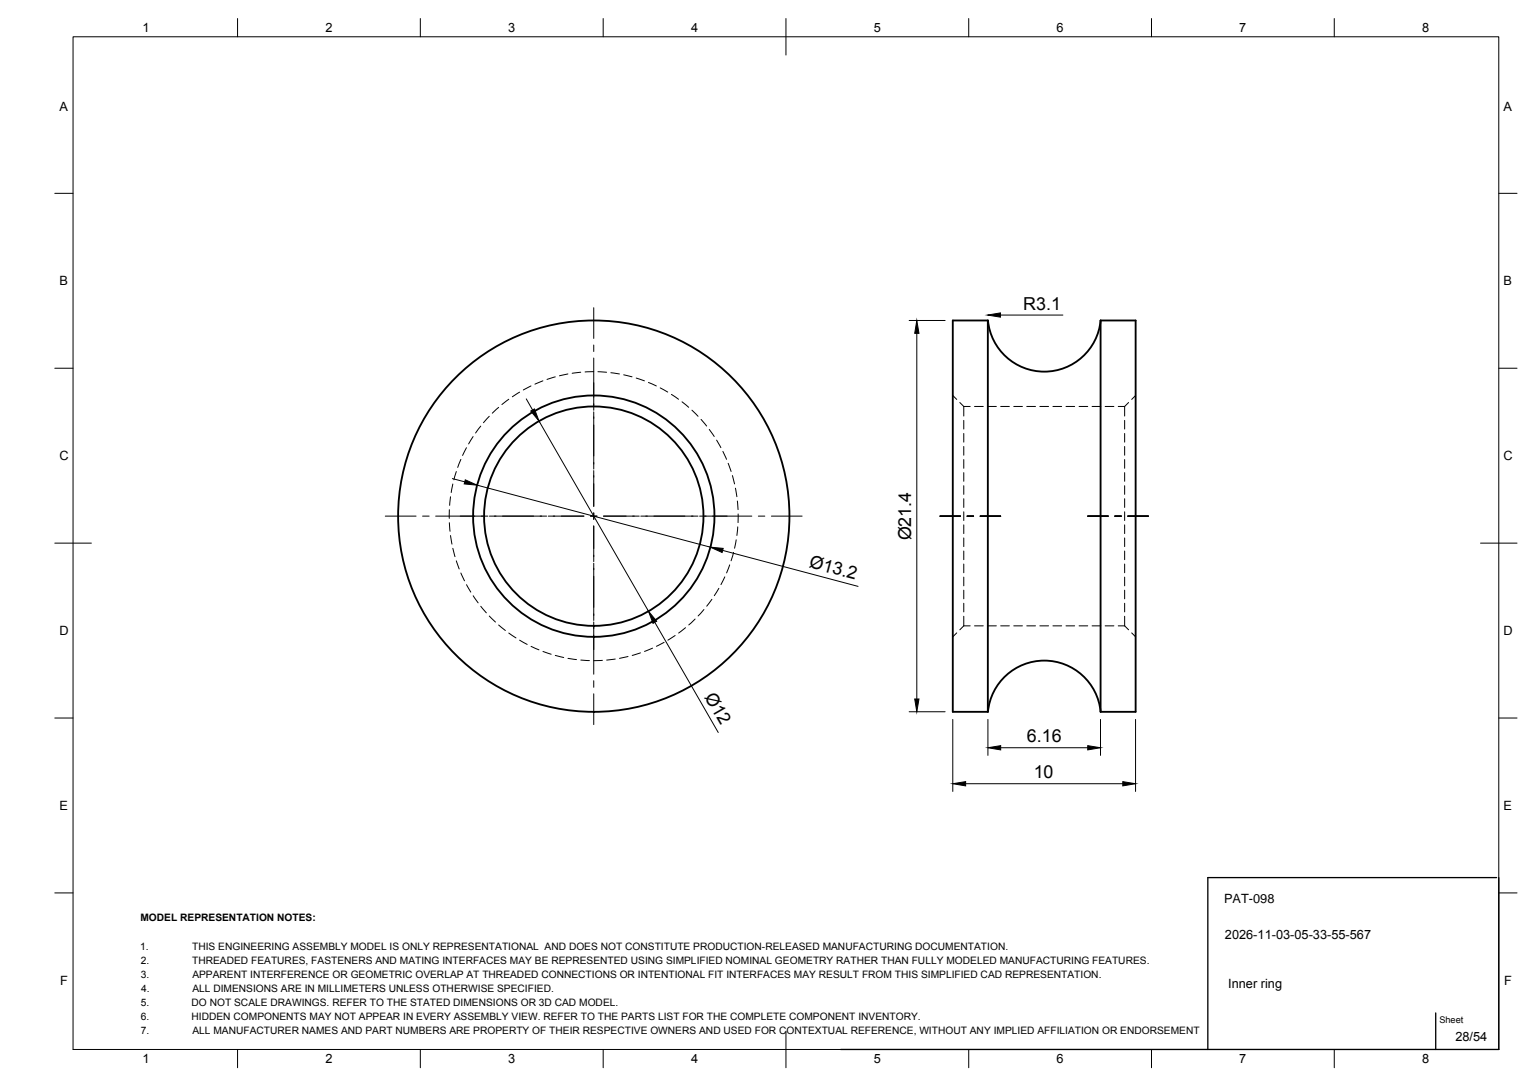
ISO-10303-21;
HEADER;
/* Generated by software containing ST-Developer
 * from STEP Tools, Inc. (www.steptools.com) 
 */

FILE_DESCRIPTION(
/* description */ ('Spring compression tester'),
/* implementation_level */ '2;1');

FILE_NAME(
/* name */ 'Inner ring.step',
/* time_stamp */ '2026-10-28T03:24:11-07:00',
/* author */ (''),
/* organization */ (''),
/* preprocessor_version */ 'ST-DEVELOPER v20.2',
/* originating_system */ 'Autodesk Translation Framework v15.17.0.0',
/* authorisation */ '');

FILE_SCHEMA (('AUTOMOTIVE_DESIGN { 1 0 10303 214 3 1 1 }'));
ENDSEC;

DATA;
#10=MECHANICAL_DESIGN_GEOMETRIC_PRESENTATION_REPRESENTATION('',(#1127),#43521);
#927=TOROIDAL_SURFACE('',#19994,1.1,0.309556);
#950=CONICAL_SURFACE('',#20005,0.63,0.785398163397448);
#951=CONICAL_SURFACE('',#20012,0.63,0.785398163397448);
#1007=SHAPE_REPRESENTATION_RELATIONSHIP('SRR','None',#43820,#1067);
#1067=ADVANCED_BREP_SHAPE_REPRESENTATION('',(#1201),#43480);
#1127=STYLED_ITEM('',(#44202),#1201);
#1201=MANIFOLD_SOLID_BREP('Body1',#18565);
#1450=FACE_BOUND('',#3851,.T.);
#1451=FACE_BOUND('',#3854,.T.);
#1888=PLANE('',#20007);
#1889=PLANE('',#20010);
#2596=FACE_OUTER_BOUND('',#3846,.T.);
#2597=FACE_OUTER_BOUND('',#3847,.T.);
#2598=FACE_OUTER_BOUND('',#3848,.T.);
#2599=FACE_OUTER_BOUND('',#3849,.T.);
#2600=FACE_OUTER_BOUND('',#3850,.T.);
#2601=FACE_OUTER_BOUND('',#3852,.T.);
#2602=FACE_OUTER_BOUND('',#3853,.T.);
#2603=FACE_OUTER_BOUND('',#3855,.T.);
#3846=EDGE_LOOP('',(#14121,#14122,#14123,#14124,#14125,#14126));
#3847=EDGE_LOOP('',(#14127,#14128,#14129,#14130,#14131));
#3848=EDGE_LOOP('',(#14132,#14133,#14134,#14135));
#3849=EDGE_LOOP('',(#14136,#14137,#14138,#14139));
#3850=EDGE_LOOP('',(#14140));
#3851=EDGE_LOOP('',(#14141));
#3852=EDGE_LOOP('',(#14142,#14143,#14144,#14145,#14146));
#3853=EDGE_LOOP('',(#14147));
#3854=EDGE_LOOP('',(#14148));
#3855=EDGE_LOOP('',(#14149,#14150,#14151,#14152));
#5301=LINE('',#28502,#6733);
#5302=LINE('',#28508,#6734);
#5303=LINE('',#28512,#6735);
#5304=LINE('',#28518,#6736);
#5305=LINE('',#28523,#6737);
#6733=VECTOR('',#23325,1.070235);
#6734=VECTOR('',#23332,0.6);
#6735=VECTOR('',#23337,0.63);
#6736=VECTOR('',#23346,1.070235);
#6737=VECTOR('',#23353,0.63);
#7727=CIRCLE('',#19995,1.070235);
#7728=CIRCLE('',#19996,1.070235);
#7729=CIRCLE('',#19997,0.309556);
#7730=CIRCLE('',#19998,1.070235);
#7731=CIRCLE('',#19999,1.070235);
#7732=CIRCLE('',#20001,1.070235);
#7733=CIRCLE('',#20003,0.6);
#7734=CIRCLE('',#20004,0.6);
#7735=CIRCLE('',#20006,0.66);
#7736=CIRCLE('',#20009,1.070235);
#7737=CIRCLE('',#20011,0.66);
#8769=VERTEX_POINT('',#28491);
#8770=VERTEX_POINT('',#28492);
#8771=VERTEX_POINT('',#28495);
#8772=VERTEX_POINT('',#28497);
#8773=VERTEX_POINT('',#28501);
#8774=VERTEX_POINT('',#28505);
#8775=VERTEX_POINT('',#28507);
#8776=VERTEX_POINT('',#28511);
#8777=VERTEX_POINT('',#28516);
#8778=VERTEX_POINT('',#28520);
#10725=EDGE_CURVE('',#8769,#8770,#7727,.T.);
#10726=EDGE_CURVE('',#8770,#8769,#7728,.T.);
#10727=EDGE_CURVE('',#8770,#8771,#7729,.T.);
#10728=EDGE_CURVE('',#8772,#8771,#7730,.T.);
#10729=EDGE_CURVE('',#8771,#8772,#7731,.T.);
#10730=EDGE_CURVE('',#8772,#8773,#5301,.T.);
#10731=EDGE_CURVE('',#8773,#8773,#7732,.T.);
#10732=EDGE_CURVE('',#8774,#8774,#7733,.T.);
#10733=EDGE_CURVE('',#8774,#8775,#5302,.T.);
#10734=EDGE_CURVE('',#8775,#8775,#7734,.T.);
#10735=EDGE_CURVE('',#8775,#8776,#5303,.T.);
#10736=EDGE_CURVE('',#8776,#8776,#7735,.T.);
#10737=EDGE_CURVE('',#8777,#8777,#7736,.T.);
#10738=EDGE_CURVE('',#8777,#8769,#5304,.T.);
#10739=EDGE_CURVE('',#8778,#8778,#7737,.T.);
#10740=EDGE_CURVE('',#8778,#8774,#5305,.T.);
#14121=ORIENTED_EDGE('',*,*,#10725,.F.);
#14122=ORIENTED_EDGE('',*,*,#10726,.F.);
#14123=ORIENTED_EDGE('',*,*,#10727,.T.);
#14124=ORIENTED_EDGE('',*,*,#10728,.F.);
#14125=ORIENTED_EDGE('',*,*,#10729,.F.);
#14126=ORIENTED_EDGE('',*,*,#10727,.F.);
#14127=ORIENTED_EDGE('',*,*,#10728,.T.);
#14128=ORIENTED_EDGE('',*,*,#10729,.T.);
#14129=ORIENTED_EDGE('',*,*,#10730,.T.);
#14130=ORIENTED_EDGE('',*,*,#10731,.T.);
#14131=ORIENTED_EDGE('',*,*,#10730,.F.);
#14132=ORIENTED_EDGE('',*,*,#10732,.T.);
#14133=ORIENTED_EDGE('',*,*,#10733,.T.);
#14134=ORIENTED_EDGE('',*,*,#10734,.F.);
#14135=ORIENTED_EDGE('',*,*,#10733,.F.);
#14136=ORIENTED_EDGE('',*,*,#10734,.T.);
#14137=ORIENTED_EDGE('',*,*,#10735,.T.);
#14138=ORIENTED_EDGE('',*,*,#10736,.F.);
#14139=ORIENTED_EDGE('',*,*,#10735,.F.);
#14140=ORIENTED_EDGE('',*,*,#10731,.F.);
#14141=ORIENTED_EDGE('',*,*,#10736,.T.);
#14142=ORIENTED_EDGE('',*,*,#10737,.F.);
#14143=ORIENTED_EDGE('',*,*,#10738,.T.);
#14144=ORIENTED_EDGE('',*,*,#10725,.T.);
#14145=ORIENTED_EDGE('',*,*,#10726,.T.);
#14146=ORIENTED_EDGE('',*,*,#10738,.F.);
#14147=ORIENTED_EDGE('',*,*,#10737,.T.);
#14148=ORIENTED_EDGE('',*,*,#10739,.F.);
#14149=ORIENTED_EDGE('',*,*,#10739,.T.);
#14150=ORIENTED_EDGE('',*,*,#10740,.T.);
#14151=ORIENTED_EDGE('',*,*,#10732,.F.);
#14152=ORIENTED_EDGE('',*,*,#10740,.F.);
#17227=CYLINDRICAL_SURFACE('',#20000,1.070235);
#17228=CYLINDRICAL_SURFACE('',#20002,0.6);
#17229=CYLINDRICAL_SURFACE('',#20008,1.070235);
#17920=ADVANCED_FACE('',(#2596),#927,.F.);
#17921=ADVANCED_FACE('',(#2597),#17227,.T.);
#17922=ADVANCED_FACE('',(#2598),#17228,.F.);
#17923=ADVANCED_FACE('',(#2599),#950,.F.);
#17924=ADVANCED_FACE('',(#2600,#1450),#1888,.T.);
#17925=ADVANCED_FACE('',(#2601),#17229,.T.);
#17926=ADVANCED_FACE('',(#2602,#1451),#1889,.T.);
#17927=ADVANCED_FACE('',(#2603),#951,.F.);
#18565=CLOSED_SHELL('',(#17920,#17921,#17922,#17923,#17924,#17925,#17926,
#17927));
#19993=AXIS2_PLACEMENT_3D('',#28489,#23309,#23310);
#19994=AXIS2_PLACEMENT_3D('',#28490,#23311,#23312);
#19995=AXIS2_PLACEMENT_3D('',#28493,#23313,#23314);
#19996=AXIS2_PLACEMENT_3D('',#28494,#23315,#23316);
#19997=AXIS2_PLACEMENT_3D('',#28496,#23317,#23318);
#19998=AXIS2_PLACEMENT_3D('',#28498,#23319,#23320);
#19999=AXIS2_PLACEMENT_3D('',#28499,#23321,#23322);
#20000=AXIS2_PLACEMENT_3D('',#28500,#23323,#23324);
#20001=AXIS2_PLACEMENT_3D('',#28503,#23326,#23327);
#20002=AXIS2_PLACEMENT_3D('',#28504,#23328,#23329);
#20003=AXIS2_PLACEMENT_3D('',#28506,#23330,#23331);
#20004=AXIS2_PLACEMENT_3D('',#28509,#23333,#23334);
#20005=AXIS2_PLACEMENT_3D('',#28510,#23335,#23336);
#20006=AXIS2_PLACEMENT_3D('',#28513,#23338,#23339);
#20007=AXIS2_PLACEMENT_3D('',#28514,#23340,#23341);
#20008=AXIS2_PLACEMENT_3D('',#28515,#23342,#23343);
#20009=AXIS2_PLACEMENT_3D('',#28517,#23344,#23345);
#20010=AXIS2_PLACEMENT_3D('',#28519,#23347,#23348);
#20011=AXIS2_PLACEMENT_3D('',#28521,#23349,#23350);
#20012=AXIS2_PLACEMENT_3D('',#28522,#23351,#23352);
#23309=DIRECTION('axis',(0.,0.,1.));
#23310=DIRECTION('refdir',(1.,0.,0.));
#23311=DIRECTION('center_axis',(0.,-1.,0.));
#23312=DIRECTION('ref_axis',(0.,0.,-1.));
#23313=DIRECTION('center_axis',(0.,-1.,0.));
#23314=DIRECTION('ref_axis',(1.,0.,0.));
#23315=DIRECTION('center_axis',(0.,-1.,0.));
#23316=DIRECTION('ref_axis',(1.,0.,0.));
#23317=DIRECTION('center_axis',(1.,0.,1.22464679914735E-16));
#23318=DIRECTION('ref_axis',(-1.22464679914735E-16,0.,1.));
#23319=DIRECTION('center_axis',(0.,1.,0.));
#23320=DIRECTION('ref_axis',(1.,0.,0.));
#23321=DIRECTION('center_axis',(0.,1.,0.));
#23322=DIRECTION('ref_axis',(1.,0.,0.));
#23323=DIRECTION('center_axis',(0.,-1.,0.));
#23324=DIRECTION('ref_axis',(1.,0.,0.));
#23325=DIRECTION('',(0.,1.,0.));
#23326=DIRECTION('center_axis',(0.,-1.,0.));
#23327=DIRECTION('ref_axis',(1.,0.,0.));
#23328=DIRECTION('center_axis',(0.,-1.,0.));
#23329=DIRECTION('ref_axis',(1.,0.,0.));
#23330=DIRECTION('center_axis',(0.,-1.,0.));
#23331=DIRECTION('ref_axis',(1.,0.,0.));
#23332=DIRECTION('',(0.,1.,0.));
#23333=DIRECTION('center_axis',(0.,-1.,0.));
#23334=DIRECTION('ref_axis',(1.,0.,0.));
#23335=DIRECTION('center_axis',(0.,1.,0.));
#23336=DIRECTION('ref_axis',(1.,0.,0.));
#23337=DIRECTION('',(-0.707106781186548,0.707106781186547,-8.65956056235493E-17));
#23338=DIRECTION('center_axis',(0.,-1.,0.));
#23339=DIRECTION('ref_axis',(1.,0.,0.));
#23340=DIRECTION('center_axis',(0.,1.,0.));
#23341=DIRECTION('ref_axis',(0.,0.,1.));
#23342=DIRECTION('center_axis',(0.,-1.,0.));
#23343=DIRECTION('ref_axis',(1.,0.,0.));
#23344=DIRECTION('center_axis',(0.,-1.,0.));
#23345=DIRECTION('ref_axis',(1.,0.,0.));
#23346=DIRECTION('',(0.,1.,0.));
#23347=DIRECTION('center_axis',(0.,-1.,0.));
#23348=DIRECTION('ref_axis',(0.,0.,-1.));
#23349=DIRECTION('center_axis',(0.,-1.,0.));
#23350=DIRECTION('ref_axis',(1.,0.,0.));
#23351=DIRECTION('center_axis',(0.,-1.,0.));
#23352=DIRECTION('ref_axis',(1.,0.,0.));
#23353=DIRECTION('',(0.707106781186548,0.707106781186547,8.65956056235493E-17));
#28489=CARTESIAN_POINT('',(0.,0.,0.));
#28490=CARTESIAN_POINT('Origin',(0.,0.,0.));
#28491=CARTESIAN_POINT('',(-1.070235,-0.308121667383195,-1.31065986708547E-16));
#28492=CARTESIAN_POINT('',(-1.31065986708547E-16,-0.308121667383195,1.070235));
#28493=CARTESIAN_POINT('Origin',(0.,-0.308121667383195,0.));
#28494=CARTESIAN_POINT('Origin',(0.,-0.308121667383195,0.));
#28495=CARTESIAN_POINT('',(-1.31065986708547E-16,0.308121667383195,1.070235));
#28496=CARTESIAN_POINT('Origin',(-1.34711147906209E-16,0.,1.1));
#28497=CARTESIAN_POINT('',(-1.070235,0.308121667383195,1.31065986708547E-16));
#28498=CARTESIAN_POINT('Origin',(0.,0.308121667383195,0.));
#28499=CARTESIAN_POINT('Origin',(0.,0.308121667383195,0.));
#28500=CARTESIAN_POINT('Origin',(0.,0.,0.));
#28501=CARTESIAN_POINT('',(-1.070235,0.5,-1.31065986708547E-16));
#28502=CARTESIAN_POINT('',(-1.070235,0.,-1.31065986708547E-16));
#28503=CARTESIAN_POINT('Origin',(0.,0.5,0.));
#28504=CARTESIAN_POINT('Origin',(0.,0.,0.));
#28505=CARTESIAN_POINT('',(-0.6,-0.44,-7.34788079488412E-17));
#28506=CARTESIAN_POINT('Origin',(0.,-0.44,0.));
#28507=CARTESIAN_POINT('',(-0.6,0.44,-7.34788079488412E-17));
#28508=CARTESIAN_POINT('',(-0.6,0.,-7.34788079488412E-17));
#28509=CARTESIAN_POINT('Origin',(0.,0.44,0.));
#28510=CARTESIAN_POINT('Origin',(0.,0.47,0.));
#28511=CARTESIAN_POINT('',(-0.66,0.5,-8.08266887437253E-17));
#28512=CARTESIAN_POINT('',(-0.63,0.47,-7.71527483462832E-17));
#28513=CARTESIAN_POINT('Origin',(0.,0.5,0.));
#28514=CARTESIAN_POINT('Origin',(1.070235,0.5,0.));
#28515=CARTESIAN_POINT('Origin',(0.,0.,0.));
#28516=CARTESIAN_POINT('',(-1.070235,-0.5,-1.31065986708547E-16));
#28517=CARTESIAN_POINT('Origin',(0.,-0.5,0.));
#28518=CARTESIAN_POINT('',(-1.070235,0.,-1.31065986708547E-16));
#28519=CARTESIAN_POINT('Origin',(0.66,-0.5,0.));
#28520=CARTESIAN_POINT('',(-0.66,-0.5,-8.08266887437253E-17));
#28521=CARTESIAN_POINT('Origin',(0.,-0.5,0.));
#28522=CARTESIAN_POINT('Origin',(0.,-0.47,0.));
#28523=CARTESIAN_POINT('',(-0.63,-0.47,-7.71527483462832E-17));
#43412=UNCERTAINTY_MEASURE_WITH_UNIT(LENGTH_MEASURE(0.001),#43522,
'DISTANCE_ACCURACY_VALUE',
'Maximum model space distance between geometric entities at asserted c
onnectivities');
#43453=UNCERTAINTY_MEASURE_WITH_UNIT(LENGTH_MEASURE(0.001),#43522,
'DISTANCE_ACCURACY_VALUE',
'Maximum model space distance between geometric entities at asserted c
onnectivities');
#43480=(
GEOMETRIC_REPRESENTATION_CONTEXT(3)
GLOBAL_UNCERTAINTY_ASSIGNED_CONTEXT((#43412))
GLOBAL_UNIT_ASSIGNED_CONTEXT((#43522,#43524,#43525))
REPRESENTATION_CONTEXT('','3D')
);
#43521=(
GEOMETRIC_REPRESENTATION_CONTEXT(3)
GLOBAL_UNCERTAINTY_ASSIGNED_CONTEXT((#43453))
GLOBAL_UNIT_ASSIGNED_CONTEXT((#43522,#43524,#43525))
REPRESENTATION_CONTEXT('','3D')
);
#43522=(
LENGTH_UNIT()
NAMED_UNIT(*)
SI_UNIT(.CENTI.,.METRE.)
);
#43524=(
NAMED_UNIT(*)
PLANE_ANGLE_UNIT()
SI_UNIT($,.RADIAN.)
);
#43525=(
NAMED_UNIT(*)
SI_UNIT($,.STERADIAN.)
SOLID_ANGLE_UNIT()
);
#43552=SHAPE_DEFINITION_REPRESENTATION(#43619,#43820);
#43619=PRODUCT_DEFINITION_SHAPE('',$,#43888);
#43820=SHAPE_REPRESENTATION('',(#19993),#43480);
#43861=PRODUCT_DEFINITION_CONTEXT('part definition',#44064,'design');
#43888=PRODUCT_DEFINITION('Inner ring','Inner ring',#43955,#43861);
#43955=PRODUCT_DEFINITION_FORMATION('',$,#44092);
#44064=APPLICATION_CONTEXT(
'Core Data for Automotive Mechanical Design Process');
#44065=PRODUCT_CONTEXT('part definition',#44064,'mechanical');
#44092=PRODUCT('Inner ring','Inner ring','Inner ring',(#44065));
#44196=COLOUR_RGB('Grey',0.48,0.52,0.57);
#44197=FILL_AREA_STYLE_COLOUR('',#44196);
#44198=FILL_AREA_STYLE('',(#44197));
#44199=SURFACE_STYLE_FILL_AREA(#44198);
#44200=SURFACE_SIDE_STYLE('',(#44199));
#44201=SURFACE_STYLE_USAGE(.BOTH.,#44200);
#44202=PRESENTATION_STYLE_ASSIGNMENT((#44201));
ENDSEC;
END-ISO-10303-21;
